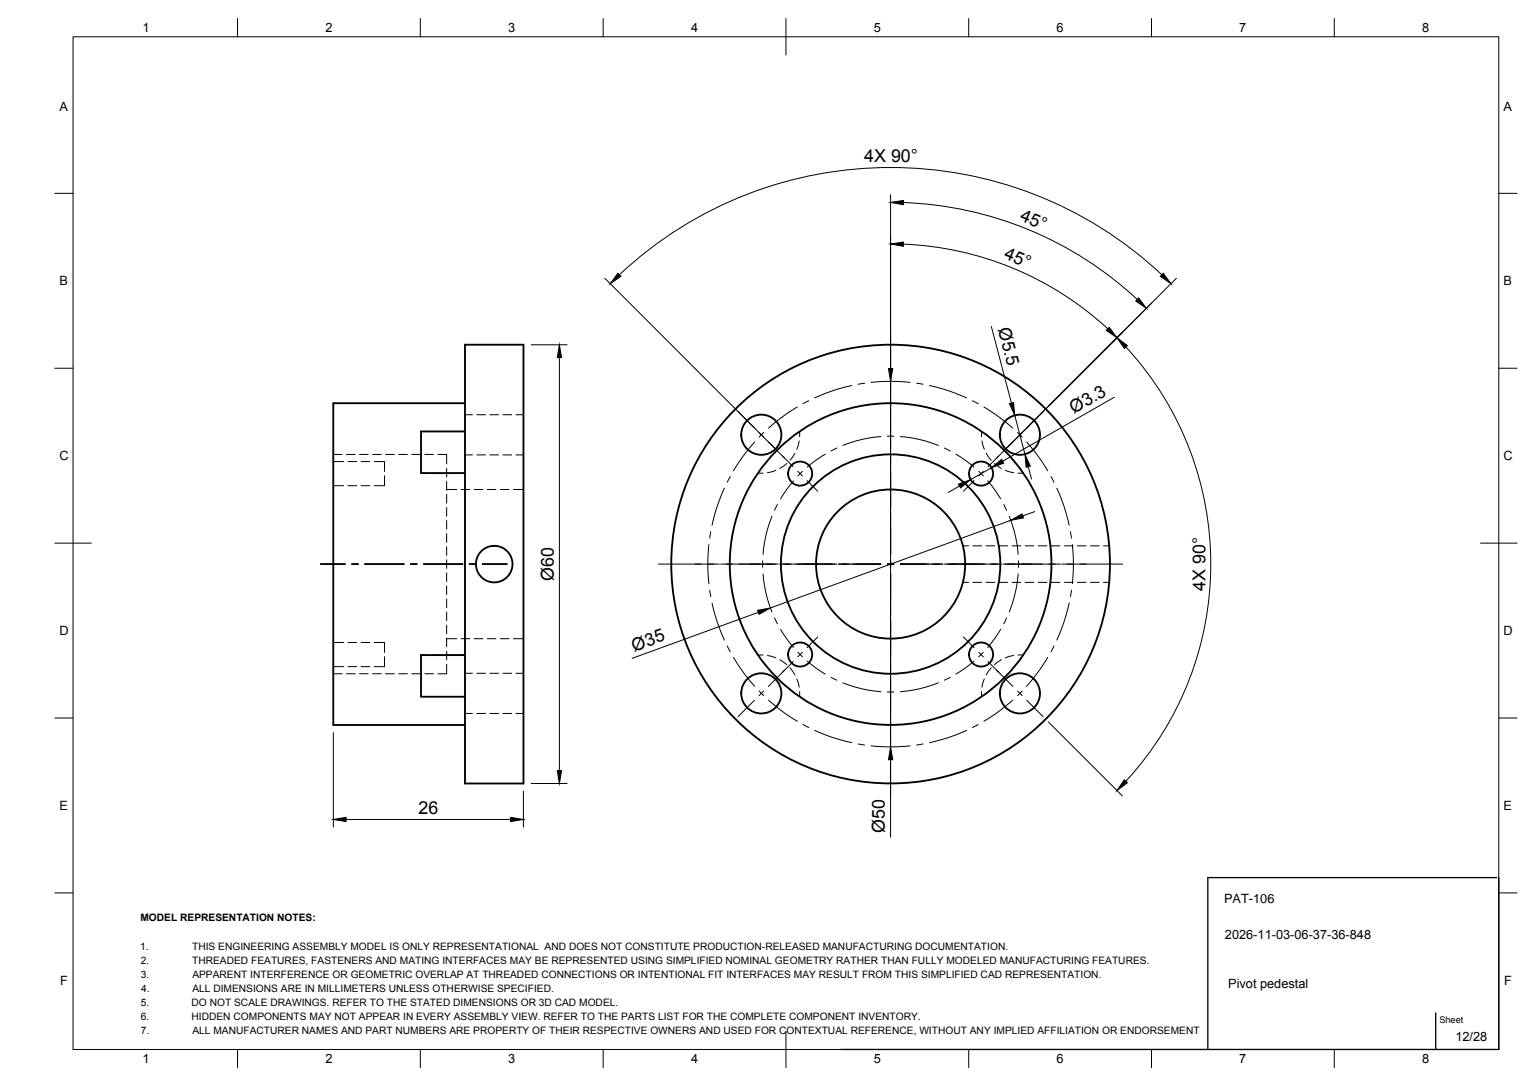
ISO-10303-21;
HEADER;
/* Generated by software containing ST-Developer
 * from STEP Tools, Inc. (www.steptools.com) 
 */

FILE_DESCRIPTION(
/* description */ ('Torsion-spring ratchet demonstrator'),
/* implementation_level */ '2;1');

FILE_NAME(
/* name */ 'Pivot pedestal.step',
/* time_stamp */ '2026-10-29T17:29:17-07:00',
/* author */ (''),
/* organization */ (''),
/* preprocessor_version */ 'ST-DEVELOPER v20.2',
/* originating_system */ 'Autodesk Translation Framework v15.17.0.0',
/* authorisation */ '');

FILE_SCHEMA (('AUTOMOTIVE_DESIGN { 1 0 10303 214 3 1 1 }'));
ENDSEC;

DATA;
#10=MECHANICAL_DESIGN_GEOMETRIC_PRESENTATION_REPRESENTATION('',(#290),#11258);
#201=B_SPLINE_CURVE_WITH_KNOTS('',3,(#7931,#7932,#7933,#7934,#7935,#7936,
#7937,#7938,#7939,#7940),.UNSPECIFIED.,.F.,.F.,(4,2,2,2,4),(0.,0.0945941824764479,
0.189188364952896,0.283770357603024,0.378352350253152),.UNSPECIFIED.);
#202=B_SPLINE_CURVE_WITH_KNOTS('',3,(#7941,#7942,#7943,#7944,#7945,#7946,
#7947,#7948,#7949,#7950,#7951,#7952,#7953,#7954,#7955,#7956,#7957,#7958,
#7959,#7960,#7961,#7962,#7963,#7964,#7965,#7966),.UNSPECIFIED.,.F.,.F.,
(4,2,2,2,2,2,2,2,2,2,2,2,4),(0.378352350253152,0.47293434290328,0.567516335553408,
0.662110518029855,0.756704700506303,0.851298882982751,0.945893065459199,
1.04047505810933,1.13505705075946,1.22963904340958,1.32422103605971,1.41881521853616,
1.51340940101261),.UNSPECIFIED.);
#203=B_SPLINE_CURVE_WITH_KNOTS('',3,(#7970,#7971,#7972,#7973,#7974,#7975,
#7976,#7977,#7978,#7979,#7980,#7981,#7982,#7983,#7984,#7985,#7986,#7987,
#7988,#7989,#7990,#7991,#7992,#7993,#7994,#7995),.UNSPECIFIED.,.F.,.F.,
(4,2,2,2,2,2,2,2,2,2,2,2,4),(0.,0.0942186410044058,0.188437282008812,0.282655768798837,
0.376874255588861,0.471092742378886,0.565311229168911,0.659529870173317,
0.753748511177723,0.847967152182129,0.942185793186535,1.03640427997656,
1.13062276676658),.UNSPECIFIED.);
#204=B_SPLINE_CURVE_WITH_KNOTS('',3,(#7996,#7997,#7998,#7999,#8000,#8001,
#8002,#8003,#8004,#8005),.UNSPECIFIED.,.F.,.F.,(4,2,2,2,4),(1.13062276676658,
1.22484125355661,1.31905974034663,1.41327838135104,1.50749702235545),
 .UNSPECIFIED.);
#242=SHAPE_REPRESENTATION_RELATIONSHIP('SRR','None',#11368,#266);
#266=ADVANCED_BREP_SHAPE_REPRESENTATION('',(#322),#11238);
#290=STYLED_ITEM('',(#11598),#322);
#322=MANIFOLD_SOLID_BREP('Body1',#5161);
#376=FACE_BOUND('',#1035,.T.);
#377=FACE_BOUND('',#1036,.T.);
#378=FACE_BOUND('',#1037,.T.);
#379=FACE_BOUND('',#1038,.T.);
#380=FACE_BOUND('',#1039,.T.);
#381=FACE_BOUND('',#1046,.T.);
#382=FACE_BOUND('',#1048,.T.);
#383=FACE_BOUND('',#1050,.T.);
#384=FACE_BOUND('',#1052,.T.);
#385=FACE_BOUND('',#1053,.T.);
#386=FACE_BOUND('',#1054,.T.);
#387=FACE_BOUND('',#1055,.T.);
#388=FACE_BOUND('',#1056,.T.);
#389=FACE_BOUND('',#1058,.T.);
#390=FACE_BOUND('',#1059,.T.);
#391=FACE_BOUND('',#1060,.T.);
#392=FACE_BOUND('',#1061,.T.);
#393=FACE_BOUND('',#1062,.T.);
#470=PLANE('',#5574);
#471=PLANE('',#5578);
#472=PLANE('',#5582);
#473=PLANE('',#5586);
#474=PLANE('',#5587);
#475=PLANE('',#5595);
#476=PLANE('',#5600);
#477=PLANE('',#5605);
#478=PLANE('',#5614);
#479=PLANE('',#5631);
#480=PLANE('',#5637);
#481=PLANE('',#5638);
#680=FACE_OUTER_BOUND('',#1016,.T.);
#681=FACE_OUTER_BOUND('',#1017,.T.);
#682=FACE_OUTER_BOUND('',#1018,.T.);
#683=FACE_OUTER_BOUND('',#1019,.T.);
#684=FACE_OUTER_BOUND('',#1020,.T.);
#685=FACE_OUTER_BOUND('',#1021,.T.);
#686=FACE_OUTER_BOUND('',#1022,.T.);
#687=FACE_OUTER_BOUND('',#1023,.T.);
#688=FACE_OUTER_BOUND('',#1024,.T.);
#689=FACE_OUTER_BOUND('',#1025,.T.);
#690=FACE_OUTER_BOUND('',#1026,.T.);
#691=FACE_OUTER_BOUND('',#1027,.T.);
#692=FACE_OUTER_BOUND('',#1028,.T.);
#693=FACE_OUTER_BOUND('',#1029,.T.);
#694=FACE_OUTER_BOUND('',#1030,.T.);
#695=FACE_OUTER_BOUND('',#1031,.T.);
#696=FACE_OUTER_BOUND('',#1032,.T.);
#697=FACE_OUTER_BOUND('',#1033,.T.);
#698=FACE_OUTER_BOUND('',#1034,.T.);
#699=FACE_OUTER_BOUND('',#1040,.T.);
#700=FACE_OUTER_BOUND('',#1041,.T.);
#701=FACE_OUTER_BOUND('',#1042,.T.);
#702=FACE_OUTER_BOUND('',#1043,.T.);
#703=FACE_OUTER_BOUND('',#1044,.T.);
#704=FACE_OUTER_BOUND('',#1045,.T.);
#705=FACE_OUTER_BOUND('',#1047,.T.);
#706=FACE_OUTER_BOUND('',#1049,.T.);
#707=FACE_OUTER_BOUND('',#1051,.T.);
#708=FACE_OUTER_BOUND('',#1057,.T.);
#1016=EDGE_LOOP('',(#3666,#3667,#3668,#3669,#3670,#3671));
#1017=EDGE_LOOP('',(#3672,#3673,#3674,#3675));
#1018=EDGE_LOOP('',(#3676));
#1019=EDGE_LOOP('',(#3677,#3678,#3679,#3680));
#1020=EDGE_LOOP('',(#3681));
#1021=EDGE_LOOP('',(#3682,#3683,#3684,#3685));
#1022=EDGE_LOOP('',(#3686));
#1023=EDGE_LOOP('',(#3687,#3688,#3689,#3690));
#1024=EDGE_LOOP('',(#3691));
#1025=EDGE_LOOP('',(#3692,#3693));
#1026=EDGE_LOOP('',(#3694,#3695,#3696,#3697));
#1027=EDGE_LOOP('',(#3698,#3699,#3700,#3701));
#1028=EDGE_LOOP('',(#3702,#3703));
#1029=EDGE_LOOP('',(#3704,#3705,#3706,#3707));
#1030=EDGE_LOOP('',(#3708,#3709));
#1031=EDGE_LOOP('',(#3710,#3711,#3712,#3713));
#1032=EDGE_LOOP('',(#3714,#3715));
#1033=EDGE_LOOP('',(#3716,#3717,#3718,#3719,#3720,#3721,#3722,#3723,#3724,
#3725,#3726,#3727,#3728,#3729,#3730,#3731,#3732,#3733,#3734,#3735));
#1034=EDGE_LOOP('',(#3736));
#1035=EDGE_LOOP('',(#3737,#3738,#3739,#3740,#3741,#3742,#3743,#3744,#3745));
#1036=EDGE_LOOP('',(#3746));
#1037=EDGE_LOOP('',(#3747));
#1038=EDGE_LOOP('',(#3748));
#1039=EDGE_LOOP('',(#3749));
#1040=EDGE_LOOP('',(#3750,#3751,#3752,#3753));
#1041=EDGE_LOOP('',(#3754,#3755,#3756,#3757));
#1042=EDGE_LOOP('',(#3758,#3759,#3760,#3761));
#1043=EDGE_LOOP('',(#3762,#3763,#3764,#3765));
#1044=EDGE_LOOP('',(#3766,#3767,#3768,#3769));
#1045=EDGE_LOOP('',(#3770));
#1046=EDGE_LOOP('',(#3771));
#1047=EDGE_LOOP('',(#3772,#3773,#3774,#3775));
#1048=EDGE_LOOP('',(#3776,#3777));
#1049=EDGE_LOOP('',(#3778,#3779,#3780,#3781));
#1050=EDGE_LOOP('',(#3782,#3783));
#1051=EDGE_LOOP('',(#3784));
#1052=EDGE_LOOP('',(#3785));
#1053=EDGE_LOOP('',(#3786));
#1054=EDGE_LOOP('',(#3787));
#1055=EDGE_LOOP('',(#3788));
#1056=EDGE_LOOP('',(#3789));
#1057=EDGE_LOOP('',(#3790));
#1058=EDGE_LOOP('',(#3791));
#1059=EDGE_LOOP('',(#3792));
#1060=EDGE_LOOP('',(#3793));
#1061=EDGE_LOOP('',(#3794));
#1062=EDGE_LOOP('',(#3795));
#1387=LINE('',#7968,#1770);
#1388=LINE('',#8010,#1771);
#1389=LINE('',#8017,#1772);
#1390=LINE('',#8024,#1773);
#1391=LINE('',#8031,#1774);
#1392=LINE('',#8041,#1775);
#1393=LINE('',#8044,#1776);
#1394=LINE('',#8048,#1777);
#1395=LINE('',#8052,#1778);
#1396=LINE('',#8059,#1779);
#1397=LINE('',#8063,#1780);
#1398=LINE('',#8070,#1781);
#1399=LINE('',#8074,#1782);
#1400=LINE('',#8082,#1783);
#1401=LINE('',#8102,#1784);
#1402=LINE('',#8106,#1785);
#1403=LINE('',#8110,#1786);
#1404=LINE('',#8114,#1787);
#1405=LINE('',#8119,#1788);
#1406=LINE('',#8126,#1789);
#1407=LINE('',#8130,#1790);
#1770=VECTOR('',#6364,0.25);
#1771=VECTOR('',#6369,0.165);
#1772=VECTOR('',#6378,0.165);
#1773=VECTOR('',#6387,0.165);
#1774=VECTOR('',#6396,0.165);
#1775=VECTOR('',#6409,1.);
#1776=VECTOR('',#6412,1.);
#1777=VECTOR('',#6415,1.);
#1778=VECTOR('',#6418,1.);
#1779=VECTOR('',#6427,1.);
#1780=VECTOR('',#6430,1.);
#1781=VECTOR('',#6439,1.);
#1782=VECTOR('',#6442,1.);
#1783=VECTOR('',#6453,2.2);
#1784=VECTOR('',#6480,0.275);
#1785=VECTOR('',#6485,0.275);
#1786=VECTOR('',#6490,0.275);
#1787=VECTOR('',#6495,0.275);
#1788=VECTOR('',#6500,1.5);
#1789=VECTOR('',#6509,3.);
#1790=VECTOR('',#6514,1.02);
#2141=CIRCLE('',#5572,0.165);
#2142=CIRCLE('',#5573,0.165);
#2143=CIRCLE('',#5576,0.165);
#2144=CIRCLE('',#5577,0.165);
#2145=CIRCLE('',#5580,0.165);
#2146=CIRCLE('',#5581,0.165);
#2147=CIRCLE('',#5584,0.165);
#2148=CIRCLE('',#5585,0.165);
#2149=CIRCLE('',#5588,2.2);
#2150=CIRCLE('',#5589,0.525);
#2151=CIRCLE('',#5591,0.525);
#2152=CIRCLE('',#5593,0.525);
#2153=CIRCLE('',#5594,0.525);
#2154=CIRCLE('',#5596,2.2);
#2155=CIRCLE('',#5598,0.525);
#2156=CIRCLE('',#5599,0.525);
#2157=CIRCLE('',#5601,2.2);
#2158=CIRCLE('',#5603,0.525);
#2159=CIRCLE('',#5604,0.525);
#2160=CIRCLE('',#5606,2.2);
#2161=CIRCLE('',#5608,2.2);
#2162=CIRCLE('',#5609,2.2);
#2163=CIRCLE('',#5610,2.2);
#2164=CIRCLE('',#5611,2.2);
#2165=CIRCLE('',#5612,2.2);
#2166=CIRCLE('',#5613,2.2);
#2167=CIRCLE('',#5615,3.);
#2168=CIRCLE('',#5616,0.275);
#2169=CIRCLE('',#5617,0.275);
#2170=CIRCLE('',#5618,0.275);
#2171=CIRCLE('',#5619,0.275);
#2172=CIRCLE('',#5621,0.275);
#2173=CIRCLE('',#5623,0.275);
#2174=CIRCLE('',#5625,0.275);
#2175=CIRCLE('',#5627,0.275);
#2176=CIRCLE('',#5629,1.5);
#2177=CIRCLE('',#5630,1.5);
#2178=CIRCLE('',#5632,1.02);
#2179=CIRCLE('',#5634,3.);
#2180=CIRCLE('',#5636,1.02);
#2409=VERTEX_POINT('',#7929);
#2410=VERTEX_POINT('',#7930);
#2411=VERTEX_POINT('',#7967);
#2412=VERTEX_POINT('',#7969);
#2413=VERTEX_POINT('',#8007);
#2414=VERTEX_POINT('',#8009);
#2415=VERTEX_POINT('',#8014);
#2416=VERTEX_POINT('',#8016);
#2417=VERTEX_POINT('',#8021);
#2418=VERTEX_POINT('',#8023);
#2419=VERTEX_POINT('',#8028);
#2420=VERTEX_POINT('',#8030);
#2421=VERTEX_POINT('',#8035);
#2422=VERTEX_POINT('',#8036);
#2423=VERTEX_POINT('',#8040);
#2424=VERTEX_POINT('',#8042);
#2425=VERTEX_POINT('',#8046);
#2426=VERTEX_POINT('',#8047);
#2427=VERTEX_POINT('',#8049);
#2428=VERTEX_POINT('',#8051);
#2429=VERTEX_POINT('',#8057);
#2430=VERTEX_POINT('',#8058);
#2431=VERTEX_POINT('',#8060);
#2432=VERTEX_POINT('',#8062);
#2433=VERTEX_POINT('',#8068);
#2434=VERTEX_POINT('',#8069);
#2435=VERTEX_POINT('',#8071);
#2436=VERTEX_POINT('',#8073);
#2437=VERTEX_POINT('',#8079);
#2438=VERTEX_POINT('',#8081);
#2439=VERTEX_POINT('',#8089);
#2440=VERTEX_POINT('',#8091);
#2441=VERTEX_POINT('',#8093);
#2442=VERTEX_POINT('',#8095);
#2443=VERTEX_POINT('',#8097);
#2444=VERTEX_POINT('',#8100);
#2445=VERTEX_POINT('',#8104);
#2446=VERTEX_POINT('',#8108);
#2447=VERTEX_POINT('',#8112);
#2448=VERTEX_POINT('',#8116);
#2449=VERTEX_POINT('',#8118);
#2450=VERTEX_POINT('',#8122);
#2451=VERTEX_POINT('',#8125);
#2452=VERTEX_POINT('',#8129);
#2893=EDGE_CURVE('',#2409,#2410,#201,.T.);
#2894=EDGE_CURVE('',#2410,#2409,#202,.T.);
#2895=EDGE_CURVE('',#2410,#2411,#1387,.T.);
#2896=EDGE_CURVE('',#2412,#2411,#203,.T.);
#2897=EDGE_CURVE('',#2411,#2412,#204,.T.);
#2898=EDGE_CURVE('',#2413,#2413,#2141,.T.);
#2899=EDGE_CURVE('',#2413,#2414,#1388,.T.);
#2900=EDGE_CURVE('',#2414,#2414,#2142,.T.);
#2901=EDGE_CURVE('',#2415,#2415,#2143,.T.);
#2902=EDGE_CURVE('',#2415,#2416,#1389,.T.);
#2903=EDGE_CURVE('',#2416,#2416,#2144,.T.);
#2904=EDGE_CURVE('',#2417,#2417,#2145,.T.);
#2905=EDGE_CURVE('',#2417,#2418,#1390,.T.);
#2906=EDGE_CURVE('',#2418,#2418,#2146,.T.);
#2907=EDGE_CURVE('',#2419,#2419,#2147,.T.);
#2908=EDGE_CURVE('',#2419,#2420,#1391,.T.);
#2909=EDGE_CURVE('',#2420,#2420,#2148,.T.);
#2910=EDGE_CURVE('',#2421,#2422,#2149,.T.);
#2911=EDGE_CURVE('',#2422,#2421,#2150,.T.);
#2912=EDGE_CURVE('',#2423,#2421,#1392,.T.);
#2913=EDGE_CURVE('',#2424,#2423,#2151,.T.);
#2914=EDGE_CURVE('',#2422,#2424,#1393,.T.);
#2915=EDGE_CURVE('',#2425,#2426,#1394,.T.);
#2916=EDGE_CURVE('',#2425,#2427,#2152,.T.);
#2917=EDGE_CURVE('',#2428,#2427,#1395,.T.);
#2918=EDGE_CURVE('',#2426,#2428,#2153,.T.);
#2919=EDGE_CURVE('',#2427,#2425,#2154,.T.);
#2920=EDGE_CURVE('',#2429,#2430,#1396,.T.);
#2921=EDGE_CURVE('',#2429,#2431,#2155,.T.);
#2922=EDGE_CURVE('',#2432,#2431,#1397,.T.);
#2923=EDGE_CURVE('',#2430,#2432,#2156,.T.);
#2924=EDGE_CURVE('',#2431,#2429,#2157,.T.);
#2925=EDGE_CURVE('',#2433,#2434,#1398,.T.);
#2926=EDGE_CURVE('',#2433,#2435,#2158,.T.);
#2927=EDGE_CURVE('',#2436,#2435,#1399,.T.);
#2928=EDGE_CURVE('',#2434,#2436,#2159,.T.);
#2929=EDGE_CURVE('',#2435,#2433,#2160,.T.);
#2930=EDGE_CURVE('',#2437,#2437,#2161,.T.);
#2931=EDGE_CURVE('',#2437,#2438,#1400,.T.);
#2932=EDGE_CURVE('',#2438,#2423,#2162,.T.);
#2933=EDGE_CURVE('',#2424,#2436,#2163,.T.);
#2934=EDGE_CURVE('',#2434,#2432,#2164,.T.);
#2935=EDGE_CURVE('',#2430,#2428,#2165,.T.);
#2936=EDGE_CURVE('',#2426,#2438,#2166,.T.);
#2937=EDGE_CURVE('',#2439,#2439,#2167,.T.);
#2938=EDGE_CURVE('',#2440,#2440,#2168,.T.);
#2939=EDGE_CURVE('',#2441,#2441,#2169,.T.);
#2940=EDGE_CURVE('',#2442,#2442,#2170,.T.);
#2941=EDGE_CURVE('',#2443,#2443,#2171,.T.);
#2942=EDGE_CURVE('',#2444,#2444,#2172,.T.);
#2943=EDGE_CURVE('',#2444,#2440,#1401,.T.);
#2944=EDGE_CURVE('',#2445,#2445,#2173,.T.);
#2945=EDGE_CURVE('',#2445,#2443,#1402,.T.);
#2946=EDGE_CURVE('',#2446,#2446,#2174,.T.);
#2947=EDGE_CURVE('',#2446,#2441,#1403,.T.);
#2948=EDGE_CURVE('',#2447,#2447,#2175,.T.);
#2949=EDGE_CURVE('',#2447,#2442,#1404,.T.);
#2950=EDGE_CURVE('',#2448,#2448,#2176,.T.);
#2951=EDGE_CURVE('',#2448,#2449,#1405,.T.);
#2952=EDGE_CURVE('',#2449,#2449,#2177,.T.);
#2953=EDGE_CURVE('',#2450,#2450,#2178,.T.);
#2954=EDGE_CURVE('',#2439,#2451,#1406,.T.);
#2955=EDGE_CURVE('',#2451,#2451,#2179,.T.);
#2956=EDGE_CURVE('',#2450,#2452,#1407,.T.);
#2957=EDGE_CURVE('',#2452,#2452,#2180,.T.);
#3666=ORIENTED_EDGE('',*,*,#2893,.F.);
#3667=ORIENTED_EDGE('',*,*,#2894,.F.);
#3668=ORIENTED_EDGE('',*,*,#2895,.T.);
#3669=ORIENTED_EDGE('',*,*,#2896,.F.);
#3670=ORIENTED_EDGE('',*,*,#2897,.F.);
#3671=ORIENTED_EDGE('',*,*,#2895,.F.);
#3672=ORIENTED_EDGE('',*,*,#2898,.F.);
#3673=ORIENTED_EDGE('',*,*,#2899,.T.);
#3674=ORIENTED_EDGE('',*,*,#2900,.F.);
#3675=ORIENTED_EDGE('',*,*,#2899,.F.);
#3676=ORIENTED_EDGE('',*,*,#2898,.T.);
#3677=ORIENTED_EDGE('',*,*,#2901,.F.);
#3678=ORIENTED_EDGE('',*,*,#2902,.T.);
#3679=ORIENTED_EDGE('',*,*,#2903,.F.);
#3680=ORIENTED_EDGE('',*,*,#2902,.F.);
#3681=ORIENTED_EDGE('',*,*,#2901,.T.);
#3682=ORIENTED_EDGE('',*,*,#2904,.F.);
#3683=ORIENTED_EDGE('',*,*,#2905,.T.);
#3684=ORIENTED_EDGE('',*,*,#2906,.F.);
#3685=ORIENTED_EDGE('',*,*,#2905,.F.);
#3686=ORIENTED_EDGE('',*,*,#2904,.T.);
#3687=ORIENTED_EDGE('',*,*,#2907,.F.);
#3688=ORIENTED_EDGE('',*,*,#2908,.T.);
#3689=ORIENTED_EDGE('',*,*,#2909,.F.);
#3690=ORIENTED_EDGE('',*,*,#2908,.F.);
#3691=ORIENTED_EDGE('',*,*,#2907,.T.);
#3692=ORIENTED_EDGE('',*,*,#2910,.F.);
#3693=ORIENTED_EDGE('',*,*,#2911,.F.);
#3694=ORIENTED_EDGE('',*,*,#2912,.F.);
#3695=ORIENTED_EDGE('',*,*,#2913,.F.);
#3696=ORIENTED_EDGE('',*,*,#2914,.F.);
#3697=ORIENTED_EDGE('',*,*,#2911,.T.);
#3698=ORIENTED_EDGE('',*,*,#2915,.F.);
#3699=ORIENTED_EDGE('',*,*,#2916,.T.);
#3700=ORIENTED_EDGE('',*,*,#2917,.F.);
#3701=ORIENTED_EDGE('',*,*,#2918,.F.);
#3702=ORIENTED_EDGE('',*,*,#2919,.F.);
#3703=ORIENTED_EDGE('',*,*,#2916,.F.);
#3704=ORIENTED_EDGE('',*,*,#2920,.F.);
#3705=ORIENTED_EDGE('',*,*,#2921,.T.);
#3706=ORIENTED_EDGE('',*,*,#2922,.F.);
#3707=ORIENTED_EDGE('',*,*,#2923,.F.);
#3708=ORIENTED_EDGE('',*,*,#2924,.F.);
#3709=ORIENTED_EDGE('',*,*,#2921,.F.);
#3710=ORIENTED_EDGE('',*,*,#2925,.F.);
#3711=ORIENTED_EDGE('',*,*,#2926,.T.);
#3712=ORIENTED_EDGE('',*,*,#2927,.F.);
#3713=ORIENTED_EDGE('',*,*,#2928,.F.);
#3714=ORIENTED_EDGE('',*,*,#2929,.F.);
#3715=ORIENTED_EDGE('',*,*,#2926,.F.);
#3716=ORIENTED_EDGE('',*,*,#2930,.F.);
#3717=ORIENTED_EDGE('',*,*,#2931,.T.);
#3718=ORIENTED_EDGE('',*,*,#2932,.T.);
#3719=ORIENTED_EDGE('',*,*,#2912,.T.);
#3720=ORIENTED_EDGE('',*,*,#2910,.T.);
#3721=ORIENTED_EDGE('',*,*,#2914,.T.);
#3722=ORIENTED_EDGE('',*,*,#2933,.T.);
#3723=ORIENTED_EDGE('',*,*,#2927,.T.);
#3724=ORIENTED_EDGE('',*,*,#2929,.T.);
#3725=ORIENTED_EDGE('',*,*,#2925,.T.);
#3726=ORIENTED_EDGE('',*,*,#2934,.T.);
#3727=ORIENTED_EDGE('',*,*,#2922,.T.);
#3728=ORIENTED_EDGE('',*,*,#2924,.T.);
#3729=ORIENTED_EDGE('',*,*,#2920,.T.);
#3730=ORIENTED_EDGE('',*,*,#2935,.T.);
#3731=ORIENTED_EDGE('',*,*,#2917,.T.);
#3732=ORIENTED_EDGE('',*,*,#2919,.T.);
#3733=ORIENTED_EDGE('',*,*,#2915,.T.);
#3734=ORIENTED_EDGE('',*,*,#2936,.T.);
#3735=ORIENTED_EDGE('',*,*,#2931,.F.);
#3736=ORIENTED_EDGE('',*,*,#2937,.T.);
#3737=ORIENTED_EDGE('',*,*,#2936,.F.);
#3738=ORIENTED_EDGE('',*,*,#2918,.T.);
#3739=ORIENTED_EDGE('',*,*,#2935,.F.);
#3740=ORIENTED_EDGE('',*,*,#2923,.T.);
#3741=ORIENTED_EDGE('',*,*,#2934,.F.);
#3742=ORIENTED_EDGE('',*,*,#2928,.T.);
#3743=ORIENTED_EDGE('',*,*,#2933,.F.);
#3744=ORIENTED_EDGE('',*,*,#2913,.T.);
#3745=ORIENTED_EDGE('',*,*,#2932,.F.);
#3746=ORIENTED_EDGE('',*,*,#2938,.T.);
#3747=ORIENTED_EDGE('',*,*,#2939,.T.);
#3748=ORIENTED_EDGE('',*,*,#2940,.T.);
#3749=ORIENTED_EDGE('',*,*,#2941,.T.);
#3750=ORIENTED_EDGE('',*,*,#2942,.F.);
#3751=ORIENTED_EDGE('',*,*,#2943,.T.);
#3752=ORIENTED_EDGE('',*,*,#2938,.F.);
#3753=ORIENTED_EDGE('',*,*,#2943,.F.);
#3754=ORIENTED_EDGE('',*,*,#2944,.F.);
#3755=ORIENTED_EDGE('',*,*,#2945,.T.);
#3756=ORIENTED_EDGE('',*,*,#2941,.F.);
#3757=ORIENTED_EDGE('',*,*,#2945,.F.);
#3758=ORIENTED_EDGE('',*,*,#2946,.F.);
#3759=ORIENTED_EDGE('',*,*,#2947,.T.);
#3760=ORIENTED_EDGE('',*,*,#2939,.F.);
#3761=ORIENTED_EDGE('',*,*,#2947,.F.);
#3762=ORIENTED_EDGE('',*,*,#2948,.F.);
#3763=ORIENTED_EDGE('',*,*,#2949,.T.);
#3764=ORIENTED_EDGE('',*,*,#2940,.F.);
#3765=ORIENTED_EDGE('',*,*,#2949,.F.);
#3766=ORIENTED_EDGE('',*,*,#2950,.F.);
#3767=ORIENTED_EDGE('',*,*,#2951,.T.);
#3768=ORIENTED_EDGE('',*,*,#2952,.F.);
#3769=ORIENTED_EDGE('',*,*,#2951,.F.);
#3770=ORIENTED_EDGE('',*,*,#2950,.T.);
#3771=ORIENTED_EDGE('',*,*,#2953,.F.);
#3772=ORIENTED_EDGE('',*,*,#2937,.F.);
#3773=ORIENTED_EDGE('',*,*,#2954,.T.);
#3774=ORIENTED_EDGE('',*,*,#2955,.T.);
#3775=ORIENTED_EDGE('',*,*,#2954,.F.);
#3776=ORIENTED_EDGE('',*,*,#2896,.T.);
#3777=ORIENTED_EDGE('',*,*,#2897,.T.);
#3778=ORIENTED_EDGE('',*,*,#2953,.T.);
#3779=ORIENTED_EDGE('',*,*,#2956,.T.);
#3780=ORIENTED_EDGE('',*,*,#2957,.T.);
#3781=ORIENTED_EDGE('',*,*,#2956,.F.);
#3782=ORIENTED_EDGE('',*,*,#2893,.T.);
#3783=ORIENTED_EDGE('',*,*,#2894,.T.);
#3784=ORIENTED_EDGE('',*,*,#2930,.T.);
#3785=ORIENTED_EDGE('',*,*,#2952,.T.);
#3786=ORIENTED_EDGE('',*,*,#2909,.T.);
#3787=ORIENTED_EDGE('',*,*,#2906,.T.);
#3788=ORIENTED_EDGE('',*,*,#2903,.T.);
#3789=ORIENTED_EDGE('',*,*,#2900,.T.);
#3790=ORIENTED_EDGE('',*,*,#2955,.F.);
#3791=ORIENTED_EDGE('',*,*,#2957,.F.);
#3792=ORIENTED_EDGE('',*,*,#2948,.T.);
#3793=ORIENTED_EDGE('',*,*,#2946,.T.);
#3794=ORIENTED_EDGE('',*,*,#2944,.T.);
#3795=ORIENTED_EDGE('',*,*,#2942,.T.);
#4788=CYLINDRICAL_SURFACE('',#5570,0.25);
#4789=CYLINDRICAL_SURFACE('',#5571,0.165);
#4790=CYLINDRICAL_SURFACE('',#5575,0.165);
#4791=CYLINDRICAL_SURFACE('',#5579,0.165);
#4792=CYLINDRICAL_SURFACE('',#5583,0.165);
#4793=CYLINDRICAL_SURFACE('',#5590,0.525);
#4794=CYLINDRICAL_SURFACE('',#5592,0.525);
#4795=CYLINDRICAL_SURFACE('',#5597,0.525);
#4796=CYLINDRICAL_SURFACE('',#5602,0.525);
#4797=CYLINDRICAL_SURFACE('',#5607,2.2);
#4798=CYLINDRICAL_SURFACE('',#5620,0.275);
#4799=CYLINDRICAL_SURFACE('',#5622,0.275);
#4800=CYLINDRICAL_SURFACE('',#5624,0.275);
#4801=CYLINDRICAL_SURFACE('',#5626,0.275);
#4802=CYLINDRICAL_SURFACE('',#5628,1.5);
#4803=CYLINDRICAL_SURFACE('',#5633,3.);
#4804=CYLINDRICAL_SURFACE('',#5635,1.02);
#4906=ADVANCED_FACE('',(#680),#4788,.F.);
#4907=ADVANCED_FACE('',(#681),#4789,.F.);
#4908=ADVANCED_FACE('',(#682),#470,.T.);
#4909=ADVANCED_FACE('',(#683),#4790,.F.);
#4910=ADVANCED_FACE('',(#684),#471,.T.);
#4911=ADVANCED_FACE('',(#685),#4791,.F.);
#4912=ADVANCED_FACE('',(#686),#472,.T.);
#4913=ADVANCED_FACE('',(#687),#4792,.F.);
#4914=ADVANCED_FACE('',(#688),#473,.T.);
#4915=ADVANCED_FACE('',(#689),#474,.F.);
#4916=ADVANCED_FACE('',(#690),#4793,.F.);
#4917=ADVANCED_FACE('',(#691),#4794,.F.);
#4918=ADVANCED_FACE('',(#692),#475,.F.);
#4919=ADVANCED_FACE('',(#693),#4795,.F.);
#4920=ADVANCED_FACE('',(#694),#476,.F.);
#4921=ADVANCED_FACE('',(#695),#4796,.F.);
#4922=ADVANCED_FACE('',(#696),#477,.F.);
#4923=ADVANCED_FACE('',(#697),#4797,.T.);
#4924=ADVANCED_FACE('',(#698,#376,#377,#378,#379,#380),#478,.T.);
#4925=ADVANCED_FACE('',(#699),#4798,.F.);
#4926=ADVANCED_FACE('',(#700),#4799,.F.);
#4927=ADVANCED_FACE('',(#701),#4800,.F.);
#4928=ADVANCED_FACE('',(#702),#4801,.F.);
#4929=ADVANCED_FACE('',(#703),#4802,.F.);
#4930=ADVANCED_FACE('',(#704,#381),#479,.T.);
#4931=ADVANCED_FACE('',(#705,#382),#4803,.T.);
#4932=ADVANCED_FACE('',(#706,#383),#4804,.F.);
#4933=ADVANCED_FACE('',(#707,#384,#385,#386,#387,#388),#480,.T.);
#4934=ADVANCED_FACE('',(#708,#389,#390,#391,#392,#393),#481,.F.);
#5161=CLOSED_SHELL('',(#4906,#4907,#4908,#4909,#4910,#4911,#4912,#4913,
#4914,#4915,#4916,#4917,#4918,#4919,#4920,#4921,#4922,#4923,#4924,#4925,
#4926,#4927,#4928,#4929,#4930,#4931,#4932,#4933,#4934));
#5569=AXIS2_PLACEMENT_3D('',#7927,#6360,#6361);
#5570=AXIS2_PLACEMENT_3D('',#7928,#6362,#6363);
#5571=AXIS2_PLACEMENT_3D('',#8006,#6365,#6366);
#5572=AXIS2_PLACEMENT_3D('',#8008,#6367,#6368);
#5573=AXIS2_PLACEMENT_3D('',#8011,#6370,#6371);
#5574=AXIS2_PLACEMENT_3D('',#8012,#6372,#6373);
#5575=AXIS2_PLACEMENT_3D('',#8013,#6374,#6375);
#5576=AXIS2_PLACEMENT_3D('',#8015,#6376,#6377);
#5577=AXIS2_PLACEMENT_3D('',#8018,#6379,#6380);
#5578=AXIS2_PLACEMENT_3D('',#8019,#6381,#6382);
#5579=AXIS2_PLACEMENT_3D('',#8020,#6383,#6384);
#5580=AXIS2_PLACEMENT_3D('',#8022,#6385,#6386);
#5581=AXIS2_PLACEMENT_3D('',#8025,#6388,#6389);
#5582=AXIS2_PLACEMENT_3D('',#8026,#6390,#6391);
#5583=AXIS2_PLACEMENT_3D('',#8027,#6392,#6393);
#5584=AXIS2_PLACEMENT_3D('',#8029,#6394,#6395);
#5585=AXIS2_PLACEMENT_3D('',#8032,#6397,#6398);
#5586=AXIS2_PLACEMENT_3D('',#8033,#6399,#6400);
#5587=AXIS2_PLACEMENT_3D('',#8034,#6401,#6402);
#5588=AXIS2_PLACEMENT_3D('',#8037,#6403,#6404);
#5589=AXIS2_PLACEMENT_3D('',#8038,#6405,#6406);
#5590=AXIS2_PLACEMENT_3D('',#8039,#6407,#6408);
#5591=AXIS2_PLACEMENT_3D('',#8043,#6410,#6411);
#5592=AXIS2_PLACEMENT_3D('',#8045,#6413,#6414);
#5593=AXIS2_PLACEMENT_3D('',#8050,#6416,#6417);
#5594=AXIS2_PLACEMENT_3D('',#8053,#6419,#6420);
#5595=AXIS2_PLACEMENT_3D('',#8054,#6421,#6422);
#5596=AXIS2_PLACEMENT_3D('',#8055,#6423,#6424);
#5597=AXIS2_PLACEMENT_3D('',#8056,#6425,#6426);
#5598=AXIS2_PLACEMENT_3D('',#8061,#6428,#6429);
#5599=AXIS2_PLACEMENT_3D('',#8064,#6431,#6432);
#5600=AXIS2_PLACEMENT_3D('',#8065,#6433,#6434);
#5601=AXIS2_PLACEMENT_3D('',#8066,#6435,#6436);
#5602=AXIS2_PLACEMENT_3D('',#8067,#6437,#6438);
#5603=AXIS2_PLACEMENT_3D('',#8072,#6440,#6441);
#5604=AXIS2_PLACEMENT_3D('',#8075,#6443,#6444);
#5605=AXIS2_PLACEMENT_3D('',#8076,#6445,#6446);
#5606=AXIS2_PLACEMENT_3D('',#8077,#6447,#6448);
#5607=AXIS2_PLACEMENT_3D('',#8078,#6449,#6450);
#5608=AXIS2_PLACEMENT_3D('',#8080,#6451,#6452);
#5609=AXIS2_PLACEMENT_3D('',#8083,#6454,#6455);
#5610=AXIS2_PLACEMENT_3D('',#8084,#6456,#6457);
#5611=AXIS2_PLACEMENT_3D('',#8085,#6458,#6459);
#5612=AXIS2_PLACEMENT_3D('',#8086,#6460,#6461);
#5613=AXIS2_PLACEMENT_3D('',#8087,#6462,#6463);
#5614=AXIS2_PLACEMENT_3D('',#8088,#6464,#6465);
#5615=AXIS2_PLACEMENT_3D('',#8090,#6466,#6467);
#5616=AXIS2_PLACEMENT_3D('',#8092,#6468,#6469);
#5617=AXIS2_PLACEMENT_3D('',#8094,#6470,#6471);
#5618=AXIS2_PLACEMENT_3D('',#8096,#6472,#6473);
#5619=AXIS2_PLACEMENT_3D('',#8098,#6474,#6475);
#5620=AXIS2_PLACEMENT_3D('',#8099,#6476,#6477);
#5621=AXIS2_PLACEMENT_3D('',#8101,#6478,#6479);
#5622=AXIS2_PLACEMENT_3D('',#8103,#6481,#6482);
#5623=AXIS2_PLACEMENT_3D('',#8105,#6483,#6484);
#5624=AXIS2_PLACEMENT_3D('',#8107,#6486,#6487);
#5625=AXIS2_PLACEMENT_3D('',#8109,#6488,#6489);
#5626=AXIS2_PLACEMENT_3D('',#8111,#6491,#6492);
#5627=AXIS2_PLACEMENT_3D('',#8113,#6493,#6494);
#5628=AXIS2_PLACEMENT_3D('',#8115,#6496,#6497);
#5629=AXIS2_PLACEMENT_3D('',#8117,#6498,#6499);
#5630=AXIS2_PLACEMENT_3D('',#8120,#6501,#6502);
#5631=AXIS2_PLACEMENT_3D('',#8121,#6503,#6504);
#5632=AXIS2_PLACEMENT_3D('',#8123,#6505,#6506);
#5633=AXIS2_PLACEMENT_3D('',#8124,#6507,#6508);
#5634=AXIS2_PLACEMENT_3D('',#8127,#6510,#6511);
#5635=AXIS2_PLACEMENT_3D('',#8128,#6512,#6513);
#5636=AXIS2_PLACEMENT_3D('',#8131,#6515,#6516);
#5637=AXIS2_PLACEMENT_3D('',#8132,#6517,#6518);
#5638=AXIS2_PLACEMENT_3D('',#8133,#6519,#6520);
#6360=DIRECTION('axis',(0.,0.,1.));
#6361=DIRECTION('refdir',(1.,0.,0.));
#6362=DIRECTION('center_axis',(1.,0.,0.));
#6363=DIRECTION('ref_axis',(0.,0.,-1.));
#6364=DIRECTION('',(1.,0.,0.));
#6365=DIRECTION('center_axis',(0.,0.,1.));
#6366=DIRECTION('ref_axis',(1.,0.,0.));
#6367=DIRECTION('center_axis',(0.,0.,1.));
#6368=DIRECTION('ref_axis',(1.,0.,0.));
#6369=DIRECTION('',(0.,0.,1.));
#6370=DIRECTION('center_axis',(0.,0.,-1.));
#6371=DIRECTION('ref_axis',(1.,0.,0.));
#6372=DIRECTION('center_axis',(0.,0.,1.));
#6373=DIRECTION('ref_axis',(1.,0.,0.));
#6374=DIRECTION('center_axis',(0.,0.,1.));
#6375=DIRECTION('ref_axis',(1.,0.,0.));
#6376=DIRECTION('center_axis',(0.,0.,1.));
#6377=DIRECTION('ref_axis',(1.,0.,0.));
#6378=DIRECTION('',(0.,0.,1.));
#6379=DIRECTION('center_axis',(0.,0.,-1.));
#6380=DIRECTION('ref_axis',(1.,0.,0.));
#6381=DIRECTION('center_axis',(0.,0.,1.));
#6382=DIRECTION('ref_axis',(1.,0.,0.));
#6383=DIRECTION('center_axis',(0.,0.,1.));
#6384=DIRECTION('ref_axis',(1.,0.,0.));
#6385=DIRECTION('center_axis',(0.,0.,1.));
#6386=DIRECTION('ref_axis',(1.,0.,0.));
#6387=DIRECTION('',(0.,0.,1.));
#6388=DIRECTION('center_axis',(0.,0.,-1.));
#6389=DIRECTION('ref_axis',(1.,0.,0.));
#6390=DIRECTION('center_axis',(0.,0.,1.));
#6391=DIRECTION('ref_axis',(1.,0.,0.));
#6392=DIRECTION('center_axis',(0.,0.,1.));
#6393=DIRECTION('ref_axis',(1.,0.,0.));
#6394=DIRECTION('center_axis',(0.,0.,1.));
#6395=DIRECTION('ref_axis',(1.,0.,0.));
#6396=DIRECTION('',(0.,0.,1.));
#6397=DIRECTION('center_axis',(0.,0.,-1.));
#6398=DIRECTION('ref_axis',(1.,0.,0.));
#6399=DIRECTION('center_axis',(0.,0.,1.));
#6400=DIRECTION('ref_axis',(1.,0.,0.));
#6401=DIRECTION('center_axis',(0.,0.,1.));
#6402=DIRECTION('ref_axis',(1.,0.,0.));
#6403=DIRECTION('center_axis',(0.,0.,1.));
#6404=DIRECTION('ref_axis',(1.,0.,0.));
#6405=DIRECTION('center_axis',(0.,0.,1.));
#6406=DIRECTION('ref_axis',(1.,0.,0.));
#6407=DIRECTION('center_axis',(0.,0.,1.));
#6408=DIRECTION('ref_axis',(1.,0.,0.));
#6409=DIRECTION('',(0.,0.,1.));
#6410=DIRECTION('center_axis',(0.,0.,1.));
#6411=DIRECTION('ref_axis',(1.,0.,0.));
#6412=DIRECTION('',(0.,0.,-1.));
#6413=DIRECTION('center_axis',(0.,0.,1.));
#6414=DIRECTION('ref_axis',(1.,0.,0.));
#6415=DIRECTION('',(0.,0.,-1.));
#6416=DIRECTION('center_axis',(0.,0.,1.));
#6417=DIRECTION('ref_axis',(1.,0.,0.));
#6418=DIRECTION('',(0.,0.,1.));
#6419=DIRECTION('center_axis',(0.,0.,1.));
#6420=DIRECTION('ref_axis',(1.,0.,0.));
#6421=DIRECTION('center_axis',(0.,0.,1.));
#6422=DIRECTION('ref_axis',(1.,0.,0.));
#6423=DIRECTION('center_axis',(0.,0.,1.));
#6424=DIRECTION('ref_axis',(1.,0.,0.));
#6425=DIRECTION('center_axis',(0.,0.,1.));
#6426=DIRECTION('ref_axis',(-0.707106781186548,-0.707106781186547,0.));
#6427=DIRECTION('',(0.,0.,-1.));
#6428=DIRECTION('center_axis',(0.,0.,1.));
#6429=DIRECTION('ref_axis',(1.,0.,0.));
#6430=DIRECTION('',(0.,0.,1.));
#6431=DIRECTION('center_axis',(0.,0.,1.));
#6432=DIRECTION('ref_axis',(1.,0.,0.));
#6433=DIRECTION('center_axis',(0.,0.,1.));
#6434=DIRECTION('ref_axis',(1.,0.,0.));
#6435=DIRECTION('center_axis',(0.,0.,1.));
#6436=DIRECTION('ref_axis',(1.,0.,0.));
#6437=DIRECTION('center_axis',(0.,0.,1.));
#6438=DIRECTION('ref_axis',(-0.707106781186547,0.707106781186548,0.));
#6439=DIRECTION('',(0.,0.,-1.));
#6440=DIRECTION('center_axis',(0.,0.,1.));
#6441=DIRECTION('ref_axis',(1.,0.,0.));
#6442=DIRECTION('',(0.,0.,1.));
#6443=DIRECTION('center_axis',(0.,0.,1.));
#6444=DIRECTION('ref_axis',(1.,0.,0.));
#6445=DIRECTION('center_axis',(0.,0.,1.));
#6446=DIRECTION('ref_axis',(1.,0.,0.));
#6447=DIRECTION('center_axis',(0.,0.,1.));
#6448=DIRECTION('ref_axis',(1.,0.,0.));
#6449=DIRECTION('center_axis',(0.,0.,1.));
#6450=DIRECTION('ref_axis',(1.,0.,0.));
#6451=DIRECTION('center_axis',(0.,0.,1.));
#6452=DIRECTION('ref_axis',(1.,0.,0.));
#6453=DIRECTION('',(0.,0.,-1.));
#6454=DIRECTION('center_axis',(0.,0.,1.));
#6455=DIRECTION('ref_axis',(1.,0.,0.));
#6456=DIRECTION('center_axis',(0.,0.,1.));
#6457=DIRECTION('ref_axis',(1.,0.,0.));
#6458=DIRECTION('center_axis',(0.,0.,1.));
#6459=DIRECTION('ref_axis',(1.,0.,0.));
#6460=DIRECTION('center_axis',(0.,0.,1.));
#6461=DIRECTION('ref_axis',(1.,0.,0.));
#6462=DIRECTION('center_axis',(0.,0.,1.));
#6463=DIRECTION('ref_axis',(1.,0.,0.));
#6464=DIRECTION('center_axis',(0.,0.,1.));
#6465=DIRECTION('ref_axis',(1.,0.,0.));
#6466=DIRECTION('center_axis',(0.,0.,1.));
#6467=DIRECTION('ref_axis',(1.,0.,0.));
#6468=DIRECTION('center_axis',(0.,0.,-1.));
#6469=DIRECTION('ref_axis',(1.,0.,0.));
#6470=DIRECTION('center_axis',(0.,0.,-1.));
#6471=DIRECTION('ref_axis',(1.,0.,0.));
#6472=DIRECTION('center_axis',(0.,0.,-1.));
#6473=DIRECTION('ref_axis',(1.,0.,0.));
#6474=DIRECTION('center_axis',(0.,0.,-1.));
#6475=DIRECTION('ref_axis',(1.,0.,0.));
#6476=DIRECTION('center_axis',(0.,0.,1.));
#6477=DIRECTION('ref_axis',(1.,0.,0.));
#6478=DIRECTION('center_axis',(0.,0.,1.));
#6479=DIRECTION('ref_axis',(1.,0.,0.));
#6480=DIRECTION('',(0.,0.,1.));
#6481=DIRECTION('center_axis',(0.,0.,1.));
#6482=DIRECTION('ref_axis',(1.,0.,0.));
#6483=DIRECTION('center_axis',(0.,0.,1.));
#6484=DIRECTION('ref_axis',(1.,0.,0.));
#6485=DIRECTION('',(0.,0.,1.));
#6486=DIRECTION('center_axis',(0.,0.,1.));
#6487=DIRECTION('ref_axis',(1.,0.,0.));
#6488=DIRECTION('center_axis',(0.,0.,1.));
#6489=DIRECTION('ref_axis',(1.,0.,0.));
#6490=DIRECTION('',(0.,0.,1.));
#6491=DIRECTION('center_axis',(0.,0.,1.));
#6492=DIRECTION('ref_axis',(1.,0.,0.));
#6493=DIRECTION('center_axis',(0.,0.,1.));
#6494=DIRECTION('ref_axis',(1.,0.,0.));
#6495=DIRECTION('',(0.,0.,1.));
#6496=DIRECTION('center_axis',(0.,0.,1.));
#6497=DIRECTION('ref_axis',(1.,0.,0.));
#6498=DIRECTION('center_axis',(0.,0.,1.));
#6499=DIRECTION('ref_axis',(1.,0.,0.));
#6500=DIRECTION('',(0.,0.,1.));
#6501=DIRECTION('center_axis',(0.,0.,-1.));
#6502=DIRECTION('ref_axis',(1.,0.,0.));
#6503=DIRECTION('center_axis',(0.,0.,1.));
#6504=DIRECTION('ref_axis',(1.,0.,0.));
#6505=DIRECTION('center_axis',(0.,0.,1.));
#6506=DIRECTION('ref_axis',(1.,0.,0.));
#6507=DIRECTION('center_axis',(0.,0.,1.));
#6508=DIRECTION('ref_axis',(1.,0.,0.));
#6509=DIRECTION('',(0.,0.,-1.));
#6510=DIRECTION('center_axis',(0.,0.,1.));
#6511=DIRECTION('ref_axis',(1.,0.,0.));
#6512=DIRECTION('center_axis',(0.,0.,1.));
#6513=DIRECTION('ref_axis',(1.,0.,0.));
#6514=DIRECTION('',(0.,0.,-1.));
#6515=DIRECTION('center_axis',(0.,0.,-1.));
#6516=DIRECTION('ref_axis',(1.,0.,0.));
#6517=DIRECTION('center_axis',(0.,0.,1.));
#6518=DIRECTION('ref_axis',(1.,0.,0.));
#6519=DIRECTION('center_axis',(0.,0.,1.));
#6520=DIRECTION('ref_axis',(1.,0.,0.));
#7927=CARTESIAN_POINT('',(0.,0.,0.));
#7928=CARTESIAN_POINT('Origin',(0.9,0.,1.4));
#7929=CARTESIAN_POINT('',(0.988888264668966,0.25,1.4));
#7930=CARTESIAN_POINT('',(1.02,-1.18386380373883E-17,1.65));
#7931=CARTESIAN_POINT('Ctrl Pts',(0.988888264668966,0.25,1.4));
#7932=CARTESIAN_POINT('Ctrl Pts',(0.988888264668966,0.25,1.43153139415882));
#7933=CARTESIAN_POINT('Ctrl Pts',(0.990553370646674,0.243672048431404,1.46507214966317));
#7934=CARTESIAN_POINT('Ctrl Pts',(0.996491737296663,0.218119830014375,1.52662620974954));
#7935=CARTESIAN_POINT('Ctrl Pts',(1.00067109353237,0.198902128206072,1.5546512623872));
#7936=CARTESIAN_POINT('Ctrl Pts',(1.00845756932386,0.154654113568716,1.59889927702456));
#7937=CARTESIAN_POINT('Ctrl Pts',(1.01258144235289,0.126627870945253,1.61811920309393));
#7938=CARTESIAN_POINT('Ctrl Pts',(1.0183917429657,0.065069600391363,1.64367304400768));
#7939=CARTESIAN_POINT('Ctrl Pts',(1.02,0.031527330883376,1.65));
#7940=CARTESIAN_POINT('Ctrl Pts',(1.02,2.77555756156289E-17,1.65));
#7941=CARTESIAN_POINT('Ctrl Pts',(1.02,6.93889390390723E-18,1.65));
#7942=CARTESIAN_POINT('Ctrl Pts',(1.02,-0.031527330883376,1.65));
#7943=CARTESIAN_POINT('Ctrl Pts',(1.0183917429657,-0.065069600391363,1.64367304400768));
#7944=CARTESIAN_POINT('Ctrl Pts',(1.01258144235289,-0.126627870945253,1.61811920309393));
#7945=CARTESIAN_POINT('Ctrl Pts',(1.00845756932386,-0.154654113568716,1.59889927702456));
#7946=CARTESIAN_POINT('Ctrl Pts',(1.00067109353237,-0.198902128206072,1.5546512623872));
#7947=CARTESIAN_POINT('Ctrl Pts',(0.996491737296663,-0.218119830014375,
1.52662620974954));
#7948=CARTESIAN_POINT('Ctrl Pts',(0.990553370646674,-0.243672048431404,
1.46507214966317));
#7949=CARTESIAN_POINT('Ctrl Pts',(0.988888264668967,-0.25,1.43153139415882));
#7950=CARTESIAN_POINT('Ctrl Pts',(0.988888264668967,-0.25,1.36846860584118));
#7951=CARTESIAN_POINT('Ctrl Pts',(0.990553370646674,-0.243672048431404,
1.33492785033683));
#7952=CARTESIAN_POINT('Ctrl Pts',(0.996491737296663,-0.218119830014375,
1.27337379025046));
#7953=CARTESIAN_POINT('Ctrl Pts',(1.00067109353237,-0.198902128206072,1.2453487376128));
#7954=CARTESIAN_POINT('Ctrl Pts',(1.00845756932386,-0.154654113568716,1.20110072297544));
#7955=CARTESIAN_POINT('Ctrl Pts',(1.01258144235289,-0.126627870945254,1.18188079690607));
#7956=CARTESIAN_POINT('Ctrl Pts',(1.0183917429657,-0.0650696003913633,1.15632695599232));
#7957=CARTESIAN_POINT('Ctrl Pts',(1.02,-0.0315273308833761,1.15));
#7958=CARTESIAN_POINT('Ctrl Pts',(1.02,0.0315273308833759,1.15));
#7959=CARTESIAN_POINT('Ctrl Pts',(1.0183917429657,0.065069600391363,1.15632695599232));
#7960=CARTESIAN_POINT('Ctrl Pts',(1.01258144235289,0.126627870945253,1.18188079690607));
#7961=CARTESIAN_POINT('Ctrl Pts',(1.00845756932386,0.154654113568716,1.20110072297544));
#7962=CARTESIAN_POINT('Ctrl Pts',(1.00067109353237,0.198902128206072,1.2453487376128));
#7963=CARTESIAN_POINT('Ctrl Pts',(0.996491737296663,0.218119830014375,1.27337379025046));
#7964=CARTESIAN_POINT('Ctrl Pts',(0.990553370646674,0.243672048431404,1.33492785033683));
#7965=CARTESIAN_POINT('Ctrl Pts',(0.988888264668967,0.25,1.36846860584118));
#7966=CARTESIAN_POINT('Ctrl Pts',(0.988888264668967,0.25,1.4));
#7967=CARTESIAN_POINT('',(3.,-3.06161699786838E-17,1.65));
#7968=CARTESIAN_POINT('',(0.9,-3.06161699786838E-17,1.65));
#7969=CARTESIAN_POINT('',(2.98956518577535,0.25,1.4));
#7970=CARTESIAN_POINT('Ctrl Pts',(2.98956518577535,0.25,1.4));
#7971=CARTESIAN_POINT('Ctrl Pts',(2.98956518577535,0.25,1.36859378633186));
#7972=CARTESIAN_POINT('Ctrl Pts',(2.99011104995181,0.24372047740942,1.33510417960069));
#7973=CARTESIAN_POINT('Ctrl Pts',(2.99208145165098,0.218202539734559,1.27351367328886));
#7974=CARTESIAN_POINT('Ctrl Pts',(2.99347740802958,0.198964922639276,1.245411532046));
#7975=CARTESIAN_POINT('Ctrl Pts',(2.99609686518216,0.154588504271054,1.20103511367778));
#7976=CARTESIAN_POINT('Ctrl Pts',(2.99749070376198,0.126486346986081,1.18179746841036));
#7977=CARTESIAN_POINT('Ctrl Pts',(2.99945625936844,0.0648957875009219,1.15627950921557));
#7978=CARTESIAN_POINT('Ctrl Pts',(3.,0.0314061622633416,1.15));
#7979=CARTESIAN_POINT('Ctrl Pts',(3.,-0.0314061622633416,1.15));
#7980=CARTESIAN_POINT('Ctrl Pts',(2.99945625936844,-0.0648957875009221,
1.15627950921557));
#7981=CARTESIAN_POINT('Ctrl Pts',(2.99749070376198,-0.126486346986081,1.18179746841036));
#7982=CARTESIAN_POINT('Ctrl Pts',(2.99609686518216,-0.154588504271054,1.20103511367778));
#7983=CARTESIAN_POINT('Ctrl Pts',(2.99347740802958,-0.198964922639276,1.245411532046));
#7984=CARTESIAN_POINT('Ctrl Pts',(2.99208145165098,-0.218202539734559,1.27351367328886));
#7985=CARTESIAN_POINT('Ctrl Pts',(2.99011104995181,-0.24372047740942,1.33510417960069));
#7986=CARTESIAN_POINT('Ctrl Pts',(2.98956518577535,-0.25,1.36859378633186));
#7987=CARTESIAN_POINT('Ctrl Pts',(2.98956518577535,-0.25,1.43140621366814));
#7988=CARTESIAN_POINT('Ctrl Pts',(2.99011104995181,-0.24372047740942,1.4648958203993));
#7989=CARTESIAN_POINT('Ctrl Pts',(2.99208145165098,-0.21820253973456,1.52648632671114));
#7990=CARTESIAN_POINT('Ctrl Pts',(2.99347740802958,-0.198964922639276,1.554588467954));
#7991=CARTESIAN_POINT('Ctrl Pts',(2.99609686518216,-0.154588504271054,1.59896488632222));
#7992=CARTESIAN_POINT('Ctrl Pts',(2.99749070376198,-0.126486346986082,1.61820253158964));
#7993=CARTESIAN_POINT('Ctrl Pts',(2.99945625936844,-0.0648957875009221,
1.64372049078443));
#7994=CARTESIAN_POINT('Ctrl Pts',(3.,-0.0314061622633417,1.65));
#7995=CARTESIAN_POINT('Ctrl Pts',(3.,-5.55111512312578E-17,1.65));
#7996=CARTESIAN_POINT('Ctrl Pts',(3.,-2.08166817117217E-17,1.65));
#7997=CARTESIAN_POINT('Ctrl Pts',(3.,0.0314061622633416,1.65));
#7998=CARTESIAN_POINT('Ctrl Pts',(2.99945625936844,0.0648957875009221,1.64372049078443));
#7999=CARTESIAN_POINT('Ctrl Pts',(2.99749070376198,0.126486346986081,1.61820253158964));
#8000=CARTESIAN_POINT('Ctrl Pts',(2.99609686518216,0.154588504271054,1.59896488632222));
#8001=CARTESIAN_POINT('Ctrl Pts',(2.99347740802958,0.198964922639276,1.554588467954));
#8002=CARTESIAN_POINT('Ctrl Pts',(2.99208145165098,0.218202539734559,1.52648632671114));
#8003=CARTESIAN_POINT('Ctrl Pts',(2.99011104995181,0.24372047740942,1.46489582039931));
#8004=CARTESIAN_POINT('Ctrl Pts',(2.98956518577535,0.25,1.43140621366814));
#8005=CARTESIAN_POINT('Ctrl Pts',(2.98956518577535,0.25,1.4));
#8006=CARTESIAN_POINT('Origin',(-1.23743686707646,-1.23743686707646,2.9));
#8007=CARTESIAN_POINT('',(-1.40243686707646,-1.23743686707646,2.9));
#8008=CARTESIAN_POINT('Origin',(-1.23743686707646,-1.23743686707646,2.9));
#8009=CARTESIAN_POINT('',(-1.40243686707646,-1.23743686707646,3.6));
#8010=CARTESIAN_POINT('',(-1.40243686707646,-1.23743686707646,2.9));
#8011=CARTESIAN_POINT('Origin',(-1.23743686707646,-1.23743686707646,3.6));
#8012=CARTESIAN_POINT('Origin',(-1.23743686707646,-1.23743686707646,2.9));
#8013=CARTESIAN_POINT('Origin',(-1.23743686707646,1.23743686707646,2.9));
#8014=CARTESIAN_POINT('',(-1.40243686707646,1.23743686707646,2.9));
#8015=CARTESIAN_POINT('Origin',(-1.23743686707646,1.23743686707646,2.9));
#8016=CARTESIAN_POINT('',(-1.40243686707646,1.23743686707646,3.6));
#8017=CARTESIAN_POINT('',(-1.40243686707646,1.23743686707646,2.9));
#8018=CARTESIAN_POINT('Origin',(-1.23743686707646,1.23743686707646,3.6));
#8019=CARTESIAN_POINT('Origin',(-1.23743686707646,1.23743686707646,2.9));
#8020=CARTESIAN_POINT('Origin',(1.23743686707646,1.23743686707646,2.9));
#8021=CARTESIAN_POINT('',(1.07243686707646,1.23743686707646,2.9));
#8022=CARTESIAN_POINT('Origin',(1.23743686707646,1.23743686707646,2.9));
#8023=CARTESIAN_POINT('',(1.07243686707646,1.23743686707646,3.6));
#8024=CARTESIAN_POINT('',(1.07243686707646,1.23743686707646,2.9));
#8025=CARTESIAN_POINT('Origin',(1.23743686707646,1.23743686707646,3.6));
#8026=CARTESIAN_POINT('Origin',(1.23743686707646,1.23743686707646,2.9));
#8027=CARTESIAN_POINT('Origin',(1.23743686707646,-1.23743686707646,2.9));
#8028=CARTESIAN_POINT('',(1.07243686707646,-1.23743686707646,2.9));
#8029=CARTESIAN_POINT('Origin',(1.23743686707646,-1.23743686707646,2.9));
#8030=CARTESIAN_POINT('',(1.07243686707646,-1.23743686707646,3.6));
#8031=CARTESIAN_POINT('',(1.07243686707646,-1.23743686707646,2.9));
#8032=CARTESIAN_POINT('Origin',(1.23743686707646,-1.23743686707646,3.6));
#8033=CARTESIAN_POINT('Origin',(1.23743686707646,-1.23743686707646,2.9));
#8034=CARTESIAN_POINT('Origin',(-1.76776695296637,-1.76776695296637,2.4));
#8035=CARTESIAN_POINT('',(-1.8139637388702,-1.24480341984751,2.4));
#8036=CARTESIAN_POINT('',(-1.24480341984751,-1.81396373887019,2.4));
#8037=CARTESIAN_POINT('Origin',(0.,0.,2.4));
#8038=CARTESIAN_POINT('Origin',(-1.76776695296637,-1.76776695296637,2.4));
#8039=CARTESIAN_POINT('Origin',(-1.76776695296637,-1.76776695296637,1.8));
#8040=CARTESIAN_POINT('',(-1.8139637388702,-1.24480341984751,1.8));
#8041=CARTESIAN_POINT('',(-1.8139637388702,-1.24480341984751,1.8));
#8042=CARTESIAN_POINT('',(-1.24480341984751,-1.81396373887019,1.8));
#8043=CARTESIAN_POINT('Origin',(-1.76776695296637,-1.76776695296637,1.8));
#8044=CARTESIAN_POINT('',(-1.24480341984751,-1.81396373887019,1.8));
#8045=CARTESIAN_POINT('Origin',(-1.76776695296637,1.76776695296637,1.8));
#8046=CARTESIAN_POINT('',(-1.81396373887019,1.24480341984751,2.4));
#8047=CARTESIAN_POINT('',(-1.81396373887019,1.24480341984751,1.8));
#8048=CARTESIAN_POINT('',(-1.81396373887019,1.24480341984751,1.8));
#8049=CARTESIAN_POINT('',(-1.24480341984751,1.81396373887019,2.4));
#8050=CARTESIAN_POINT('Origin',(-1.76776695296637,1.76776695296637,2.4));
#8051=CARTESIAN_POINT('',(-1.24480341984751,1.81396373887019,1.8));
#8052=CARTESIAN_POINT('',(-1.24480341984751,1.81396373887019,1.8));
#8053=CARTESIAN_POINT('Origin',(-1.76776695296637,1.76776695296637,1.8));
#8054=CARTESIAN_POINT('Origin',(-1.76776695296637,1.76776695296637,2.4));
#8055=CARTESIAN_POINT('Origin',(0.,0.,2.4));
#8056=CARTESIAN_POINT('Origin',(1.76776695296637,1.76776695296637,1.8));
#8057=CARTESIAN_POINT('',(1.24480341984751,1.81396373887019,2.4));
#8058=CARTESIAN_POINT('',(1.24480341984751,1.81396373887019,1.8));
#8059=CARTESIAN_POINT('',(1.24480341984751,1.81396373887019,1.8));
#8060=CARTESIAN_POINT('',(1.81396373887019,1.24480341984751,2.4));
#8061=CARTESIAN_POINT('Origin',(1.76776695296637,1.76776695296637,2.4));
#8062=CARTESIAN_POINT('',(1.81396373887019,1.24480341984751,1.8));
#8063=CARTESIAN_POINT('',(1.81396373887019,1.24480341984751,1.8));
#8064=CARTESIAN_POINT('Origin',(1.76776695296637,1.76776695296637,1.8));
#8065=CARTESIAN_POINT('Origin',(1.76776695296637,1.76776695296637,2.4));
#8066=CARTESIAN_POINT('Origin',(0.,0.,2.4));
#8067=CARTESIAN_POINT('Origin',(1.76776695296637,-1.76776695296637,1.8));
#8068=CARTESIAN_POINT('',(1.81396373887019,-1.24480341984751,2.4));
#8069=CARTESIAN_POINT('',(1.81396373887019,-1.24480341984751,1.8));
#8070=CARTESIAN_POINT('',(1.81396373887019,-1.24480341984751,1.8));
#8071=CARTESIAN_POINT('',(1.24480341984751,-1.8139637388702,2.4));
#8072=CARTESIAN_POINT('Origin',(1.76776695296637,-1.76776695296637,2.4));
#8073=CARTESIAN_POINT('',(1.24480341984751,-1.8139637388702,1.8));
#8074=CARTESIAN_POINT('',(1.24480341984751,-1.8139637388702,1.8));
#8075=CARTESIAN_POINT('Origin',(1.76776695296637,-1.76776695296637,1.8));
#8076=CARTESIAN_POINT('Origin',(1.76776695296637,-1.76776695296637,2.4));
#8077=CARTESIAN_POINT('Origin',(0.,0.,2.4));
#8078=CARTESIAN_POINT('Origin',(0.,0.,1.));
#8079=CARTESIAN_POINT('',(-2.2,-2.69422295812418E-16,3.6));
#8080=CARTESIAN_POINT('Origin',(0.,0.,3.6));
#8081=CARTESIAN_POINT('',(-2.2,-2.69422295812418E-16,1.8));
#8082=CARTESIAN_POINT('',(-2.2,-2.69422295812418E-16,1.));
#8083=CARTESIAN_POINT('Origin',(0.,0.,1.8));
#8084=CARTESIAN_POINT('Origin',(0.,0.,1.8));
#8085=CARTESIAN_POINT('Origin',(0.,0.,1.8));
#8086=CARTESIAN_POINT('Origin',(0.,0.,1.8));
#8087=CARTESIAN_POINT('Origin',(0.,0.,1.8));
#8088=CARTESIAN_POINT('Origin',(0.,0.,1.8));
#8089=CARTESIAN_POINT('',(-3.,-3.67394039744206E-16,1.8));
#8090=CARTESIAN_POINT('Origin',(0.,0.,1.8));
#8091=CARTESIAN_POINT('',(-2.04276695296637,-1.76776695296637,1.8));
#8092=CARTESIAN_POINT('Origin',(-1.76776695296637,-1.76776695296637,1.8));
#8093=CARTESIAN_POINT('',(1.49276695296637,1.76776695296637,1.8));
#8094=CARTESIAN_POINT('Origin',(1.76776695296637,1.76776695296637,1.8));
#8095=CARTESIAN_POINT('',(1.49276695296637,-1.76776695296637,1.8));
#8096=CARTESIAN_POINT('Origin',(1.76776695296637,-1.76776695296637,1.8));
#8097=CARTESIAN_POINT('',(-2.04276695296637,1.76776695296637,1.8));
#8098=CARTESIAN_POINT('Origin',(-1.76776695296637,1.76776695296637,1.8));
#8099=CARTESIAN_POINT('Origin',(-1.76776695296637,-1.76776695296637,0.9));
#8100=CARTESIAN_POINT('',(-2.04276695296637,-1.76776695296637,1.));
#8101=CARTESIAN_POINT('Origin',(-1.76776695296637,-1.76776695296637,1.));
#8102=CARTESIAN_POINT('',(-2.04276695296637,-1.76776695296637,0.9));
#8103=CARTESIAN_POINT('Origin',(-1.76776695296637,1.76776695296637,0.9));
#8104=CARTESIAN_POINT('',(-2.04276695296637,1.76776695296637,1.));
#8105=CARTESIAN_POINT('Origin',(-1.76776695296637,1.76776695296637,1.));
#8106=CARTESIAN_POINT('',(-2.04276695296637,1.76776695296637,0.9));
#8107=CARTESIAN_POINT('Origin',(1.76776695296637,1.76776695296637,0.9));
#8108=CARTESIAN_POINT('',(1.49276695296637,1.76776695296637,1.));
#8109=CARTESIAN_POINT('Origin',(1.76776695296637,1.76776695296637,1.));
#8110=CARTESIAN_POINT('',(1.49276695296637,1.76776695296637,0.9));
#8111=CARTESIAN_POINT('Origin',(1.76776695296637,-1.76776695296637,0.9));
#8112=CARTESIAN_POINT('',(1.49276695296637,-1.76776695296637,1.));
#8113=CARTESIAN_POINT('Origin',(1.76776695296637,-1.76776695296637,1.));
#8114=CARTESIAN_POINT('',(1.49276695296637,-1.76776695296637,0.9));
#8115=CARTESIAN_POINT('Origin',(0.,0.,2.05));
#8116=CARTESIAN_POINT('',(-1.5,-1.83697019872103E-16,2.05));
#8117=CARTESIAN_POINT('Origin',(0.,0.,2.05));
#8118=CARTESIAN_POINT('',(-1.5,1.83697019872103E-16,3.6));
#8119=CARTESIAN_POINT('',(-1.5,-1.83697019872103E-16,2.05));
#8120=CARTESIAN_POINT('Origin',(0.,0.,3.6));
#8121=CARTESIAN_POINT('Origin',(0.,0.,2.05));
#8122=CARTESIAN_POINT('',(-1.02,-1.2491397351303E-16,2.05));
#8123=CARTESIAN_POINT('Origin',(0.,0.,2.05));
#8124=CARTESIAN_POINT('Origin',(0.,0.,1.));
#8125=CARTESIAN_POINT('',(-3.,-3.67394039744206E-16,1.));
#8126=CARTESIAN_POINT('',(-3.,-3.67394039744206E-16,1.));
#8127=CARTESIAN_POINT('Origin',(0.,0.,1.));
#8128=CARTESIAN_POINT('Origin',(0.,0.,1.));
#8129=CARTESIAN_POINT('',(-1.02,-1.2491397351303E-16,1.));
#8130=CARTESIAN_POINT('',(-1.02,-1.2491397351303E-16,1.));
#8131=CARTESIAN_POINT('Origin',(0.,0.,1.));
#8132=CARTESIAN_POINT('Origin',(0.,0.,3.6));
#8133=CARTESIAN_POINT('Origin',(0.,0.,1.));
#11208=UNCERTAINTY_MEASURE_WITH_UNIT(LENGTH_MEASURE(0.001),#11259,
'DISTANCE_ACCURACY_VALUE',
'Maximum model space distance between geometric entities at asserted c
onnectivities');
#11228=UNCERTAINTY_MEASURE_WITH_UNIT(LENGTH_MEASURE(0.001),#11259,
'DISTANCE_ACCURACY_VALUE',
'Maximum model space distance between geometric entities at asserted c
onnectivities');
#11238=(
GEOMETRIC_REPRESENTATION_CONTEXT(3)
GLOBAL_UNCERTAINTY_ASSIGNED_CONTEXT((#11208))
GLOBAL_UNIT_ASSIGNED_CONTEXT((#11259,#11261,#11262))
REPRESENTATION_CONTEXT('','3D')
);
#11258=(
GEOMETRIC_REPRESENTATION_CONTEXT(3)
GLOBAL_UNCERTAINTY_ASSIGNED_CONTEXT((#11228))
GLOBAL_UNIT_ASSIGNED_CONTEXT((#11259,#11261,#11262))
REPRESENTATION_CONTEXT('','3D')
);
#11259=(
LENGTH_UNIT()
NAMED_UNIT(*)
SI_UNIT(.CENTI.,.METRE.)
);
#11261=(
NAMED_UNIT(*)
PLANE_ANGLE_UNIT()
SI_UNIT($,.RADIAN.)
);
#11262=(
NAMED_UNIT(*)
SI_UNIT($,.STERADIAN.)
SOLID_ANGLE_UNIT()
);
#11272=SHAPE_DEFINITION_REPRESENTATION(#11301,#11368);
#11301=PRODUCT_DEFINITION_SHAPE('',$,#11398);
#11368=SHAPE_REPRESENTATION('',(#5569),#11238);
#11388=PRODUCT_DEFINITION_CONTEXT('part definition',#11477,'design');
#11398=PRODUCT_DEFINITION('Pivot pedestal','Pivot pedestal',#11427,#11388);
#11427=PRODUCT_DEFINITION_FORMATION('',$,#11488);
#11477=APPLICATION_CONTEXT(
'Core Data for Automotive Mechanical Design Process');
#11478=PRODUCT_CONTEXT('part definition',#11477,'mechanical');
#11488=PRODUCT('Pivot pedestal','Pivot pedestal','Pivot pedestal',(#11478));
#11592=COLOUR_RGB('Off White',0.89,0.88,0.83);
#11593=FILL_AREA_STYLE_COLOUR('',#11592);
#11594=FILL_AREA_STYLE('',(#11593));
#11595=SURFACE_STYLE_FILL_AREA(#11594);
#11596=SURFACE_SIDE_STYLE('',(#11595));
#11597=SURFACE_STYLE_USAGE(.BOTH.,#11596);
#11598=PRESENTATION_STYLE_ASSIGNMENT((#11597));
ENDSEC;
END-ISO-10303-21;
